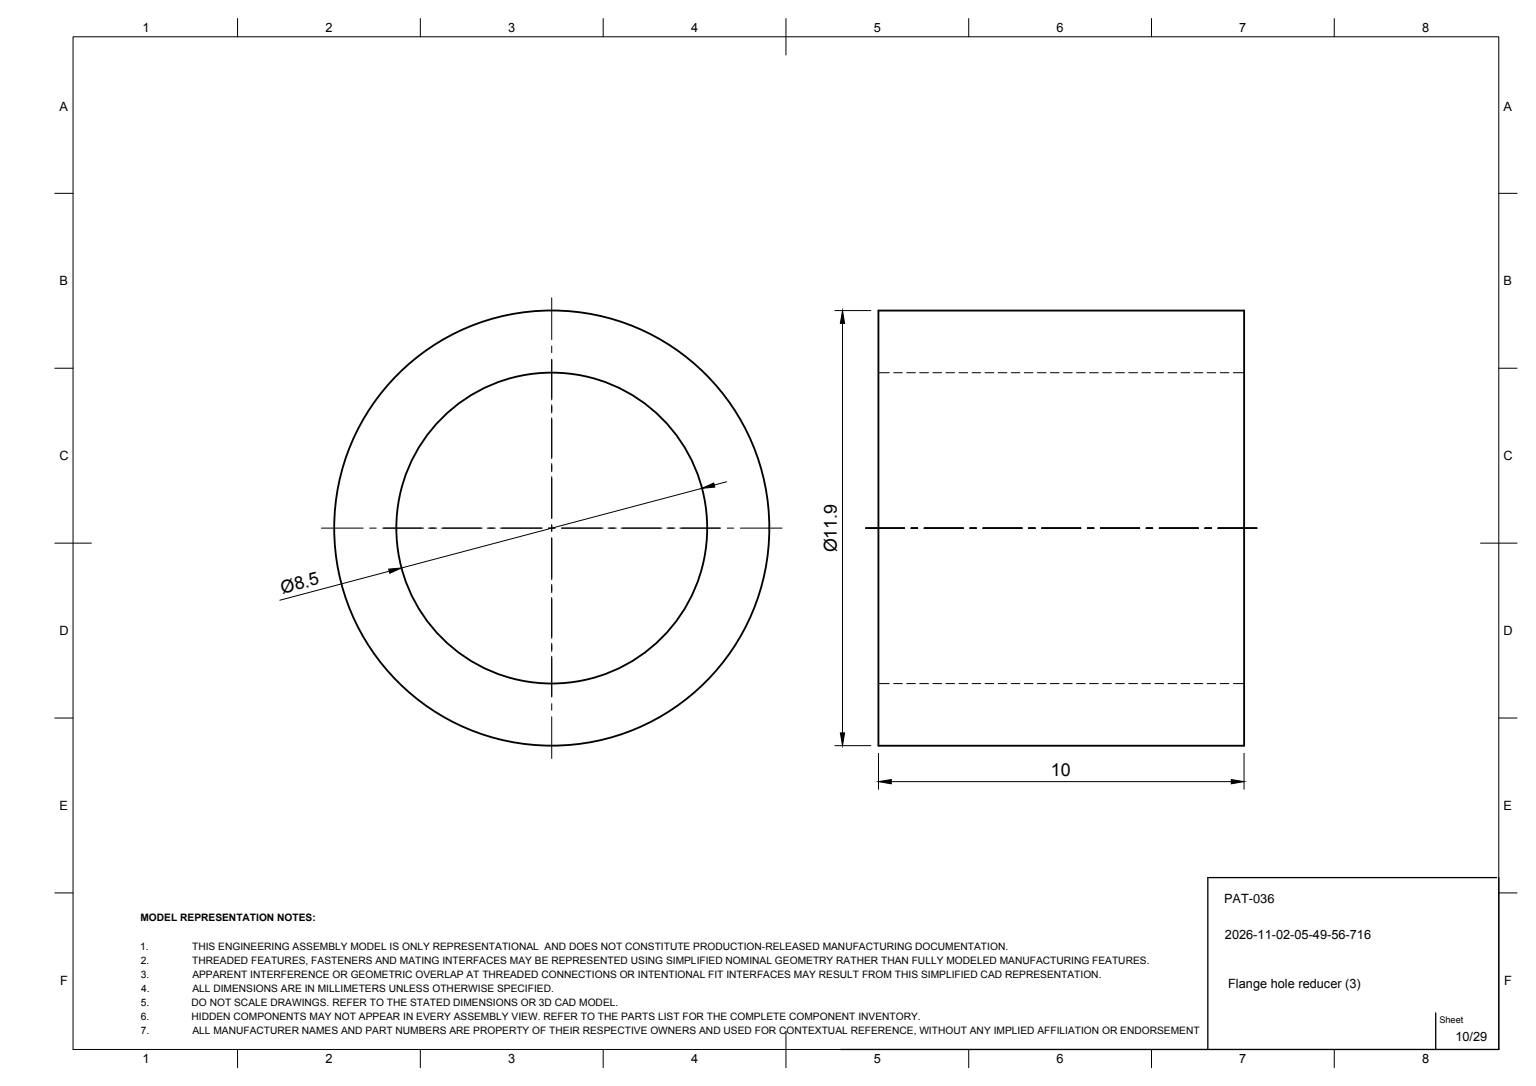
ISO-10303-21;
HEADER;
/* Generated by software containing ST-Developer
 * from STEP Tools, Inc. (www.steptools.com) 
 */

FILE_DESCRIPTION(
/* description */ ('Flange-mounted spindle'),
/* implementation_level */ '2;1');

FILE_NAME(
/* name */ 'Flange hole reducer (3).step',
/* time_stamp */ '2026-10-27T10:49:51-07:00',
/* author */ (''),
/* organization */ (''),
/* preprocessor_version */ 'ST-DEVELOPER v20.2',
/* originating_system */ 'Autodesk Translation Framework v15.17.0.0',
/* authorisation */ '');

FILE_SCHEMA (('AUTOMOTIVE_DESIGN { 1 0 10303 214 3 1 1 }'));
ENDSEC;

DATA;
#10=MECHANICAL_DESIGN_GEOMETRIC_PRESENTATION_REPRESENTATION('',(#343),#11764);
#289=SHAPE_REPRESENTATION_RELATIONSHIP('SRR','None',#11885,#316);
#316=ADVANCED_BREP_SHAPE_REPRESENTATION('',(#371),#11740);
#343=STYLED_ITEM('',(#12113),#371);
#371=MANIFOLD_SOLID_BREP('Body1',#6135);
#415=FACE_BOUND('',#1081,.T.);
#416=FACE_BOUND('',#1083,.T.);
#526=PLANE('',#6538);
#527=PLANE('',#6539);
#709=FACE_OUTER_BOUND('',#1078,.T.);
#710=FACE_OUTER_BOUND('',#1079,.T.);
#711=FACE_OUTER_BOUND('',#1080,.T.);
#712=FACE_OUTER_BOUND('',#1082,.T.);
#1078=EDGE_LOOP('',(#4155,#4156,#4157,#4158));
#1079=EDGE_LOOP('',(#4159,#4160,#4161,#4162));
#1080=EDGE_LOOP('',(#4163));
#1081=EDGE_LOOP('',(#4164));
#1082=EDGE_LOOP('',(#4165));
#1083=EDGE_LOOP('',(#4166));
#1524=LINE('',#9300,#1946);
#1525=LINE('',#9306,#1947);
#1946=VECTOR('',#7403,0.425);
#1947=VECTOR('',#7410,0.595);
#2353=CIRCLE('',#6533,0.425);
#2354=CIRCLE('',#6534,0.425);
#2355=CIRCLE('',#6536,0.595);
#2356=CIRCLE('',#6537,0.595);
#2699=VERTEX_POINT('',#9297);
#2700=VERTEX_POINT('',#9299);
#2701=VERTEX_POINT('',#9303);
#2702=VERTEX_POINT('',#9305);
#3270=EDGE_CURVE('',#2699,#2699,#2353,.T.);
#3271=EDGE_CURVE('',#2699,#2700,#1524,.T.);
#3272=EDGE_CURVE('',#2700,#2700,#2354,.T.);
#3273=EDGE_CURVE('',#2701,#2701,#2355,.T.);
#3274=EDGE_CURVE('',#2701,#2702,#1525,.T.);
#3275=EDGE_CURVE('',#2702,#2702,#2356,.T.);
#4155=ORIENTED_EDGE('',*,*,#3270,.F.);
#4156=ORIENTED_EDGE('',*,*,#3271,.T.);
#4157=ORIENTED_EDGE('',*,*,#3272,.T.);
#4158=ORIENTED_EDGE('',*,*,#3271,.F.);
#4159=ORIENTED_EDGE('',*,*,#3273,.F.);
#4160=ORIENTED_EDGE('',*,*,#3274,.T.);
#4161=ORIENTED_EDGE('',*,*,#3275,.T.);
#4162=ORIENTED_EDGE('',*,*,#3274,.F.);
#4163=ORIENTED_EDGE('',*,*,#3273,.T.);
#4164=ORIENTED_EDGE('',*,*,#3270,.T.);
#4165=ORIENTED_EDGE('',*,*,#3275,.F.);
#4166=ORIENTED_EDGE('',*,*,#3272,.F.);
#5640=CYLINDRICAL_SURFACE('',#6532,0.425);
#5641=CYLINDRICAL_SURFACE('',#6535,0.595);
#5820=ADVANCED_FACE('',(#709),#5640,.F.);
#5821=ADVANCED_FACE('',(#710),#5641,.T.);
#5822=ADVANCED_FACE('',(#711,#415),#526,.T.);
#5823=ADVANCED_FACE('',(#712,#416),#527,.F.);
#6135=CLOSED_SHELL('',(#5820,#5821,#5822,#5823));
#6531=AXIS2_PLACEMENT_3D('',#9295,#7397,#7398);
#6532=AXIS2_PLACEMENT_3D('',#9296,#7399,#7400);
#6533=AXIS2_PLACEMENT_3D('',#9298,#7401,#7402);
#6534=AXIS2_PLACEMENT_3D('',#9301,#7404,#7405);
#6535=AXIS2_PLACEMENT_3D('',#9302,#7406,#7407);
#6536=AXIS2_PLACEMENT_3D('',#9304,#7408,#7409);
#6537=AXIS2_PLACEMENT_3D('',#9307,#7411,#7412);
#6538=AXIS2_PLACEMENT_3D('',#9308,#7413,#7414);
#6539=AXIS2_PLACEMENT_3D('',#9309,#7415,#7416);
#7397=DIRECTION('axis',(0.,0.,1.));
#7398=DIRECTION('refdir',(1.,0.,0.));
#7399=DIRECTION('center_axis',(0.,1.,0.));
#7400=DIRECTION('ref_axis',(1.,0.,0.));
#7401=DIRECTION('center_axis',(0.,-1.,0.));
#7402=DIRECTION('ref_axis',(1.,0.,0.));
#7403=DIRECTION('',(0.,-1.,0.));
#7404=DIRECTION('center_axis',(0.,-1.,0.));
#7405=DIRECTION('ref_axis',(1.,0.,0.));
#7406=DIRECTION('center_axis',(0.,1.,0.));
#7407=DIRECTION('ref_axis',(1.,0.,0.));
#7408=DIRECTION('center_axis',(0.,1.,0.));
#7409=DIRECTION('ref_axis',(1.,0.,0.));
#7410=DIRECTION('',(0.,-1.,0.));
#7411=DIRECTION('center_axis',(0.,1.,0.));
#7412=DIRECTION('ref_axis',(1.,0.,0.));
#7413=DIRECTION('center_axis',(0.,1.,0.));
#7414=DIRECTION('ref_axis',(1.,0.,0.));
#7415=DIRECTION('center_axis',(0.,1.,0.));
#7416=DIRECTION('ref_axis',(1.,0.,0.));
#9295=CARTESIAN_POINT('',(0.,0.,0.));
#9296=CARTESIAN_POINT('Origin',(3.2,-0.5,11.2));
#9297=CARTESIAN_POINT('',(2.775,0.5,11.2));
#9298=CARTESIAN_POINT('Origin',(3.2,0.5,11.2));
#9299=CARTESIAN_POINT('',(2.775,-0.5,11.2));
#9300=CARTESIAN_POINT('',(2.775,-0.5,11.2));
#9301=CARTESIAN_POINT('Origin',(3.2,-0.5,11.2));
#9302=CARTESIAN_POINT('Origin',(3.2,-0.5,11.2));
#9303=CARTESIAN_POINT('',(2.605,0.5,11.2));
#9304=CARTESIAN_POINT('Origin',(3.2,0.5,11.2));
#9305=CARTESIAN_POINT('',(2.605,-0.5,11.2));
#9306=CARTESIAN_POINT('',(2.605,-0.5,11.2));
#9307=CARTESIAN_POINT('Origin',(3.2,-0.5,11.2));
#9308=CARTESIAN_POINT('Origin',(3.2,0.5,11.2));
#9309=CARTESIAN_POINT('Origin',(3.2,-0.5,11.2));
#11708=UNCERTAINTY_MEASURE_WITH_UNIT(LENGTH_MEASURE(0.001),#11765,
'DISTANCE_ACCURACY_VALUE',
'Maximum model space distance between geometric entities at asserted c
onnectivities');
#11732=UNCERTAINTY_MEASURE_WITH_UNIT(LENGTH_MEASURE(0.001),#11765,
'DISTANCE_ACCURACY_VALUE',
'Maximum model space distance between geometric entities at asserted c
onnectivities');
#11740=(
GEOMETRIC_REPRESENTATION_CONTEXT(3)
GLOBAL_UNCERTAINTY_ASSIGNED_CONTEXT((#11708))
GLOBAL_UNIT_ASSIGNED_CONTEXT((#11765,#11767,#11768))
REPRESENTATION_CONTEXT('','3D')
);
#11764=(
GEOMETRIC_REPRESENTATION_CONTEXT(3)
GLOBAL_UNCERTAINTY_ASSIGNED_CONTEXT((#11732))
GLOBAL_UNIT_ASSIGNED_CONTEXT((#11765,#11767,#11768))
REPRESENTATION_CONTEXT('','3D')
);
#11765=(
LENGTH_UNIT()
NAMED_UNIT(*)
SI_UNIT(.CENTI.,.METRE.)
);
#11767=(
NAMED_UNIT(*)
PLANE_ANGLE_UNIT()
SI_UNIT($,.RADIAN.)
);
#11768=(
NAMED_UNIT(*)
SI_UNIT($,.STERADIAN.)
SOLID_ANGLE_UNIT()
);
#11776=SHAPE_DEFINITION_REPRESENTATION(#11807,#11885);
#11807=PRODUCT_DEFINITION_SHAPE('',$,#11917);
#11885=SHAPE_REPRESENTATION('',(#6531),#11740);
#11909=PRODUCT_DEFINITION_CONTEXT('part definition',#12004,'design');
#11917=PRODUCT_DEFINITION('Flange hole reducer (3)',
'Flange hole reducer (3)',#11948,#11909);
#11948=PRODUCT_DEFINITION_FORMATION('',$,#12013);
#12004=APPLICATION_CONTEXT(
'Core Data for Automotive Mechanical Design Process');
#12005=PRODUCT_CONTEXT('part definition',#12004,'mechanical');
#12013=PRODUCT('Flange hole reducer (3)','Flange hole reducer (3)',
'Flange hole reducer (3)',(#12005));
#12107=COLOUR_RGB('Off White',0.89,0.88,0.83);
#12108=FILL_AREA_STYLE_COLOUR('',#12107);
#12109=FILL_AREA_STYLE('',(#12108));
#12110=SURFACE_STYLE_FILL_AREA(#12109);
#12111=SURFACE_SIDE_STYLE('',(#12110));
#12112=SURFACE_STYLE_USAGE(.BOTH.,#12111);
#12113=PRESENTATION_STYLE_ASSIGNMENT((#12112));
ENDSEC;
END-ISO-10303-21;
